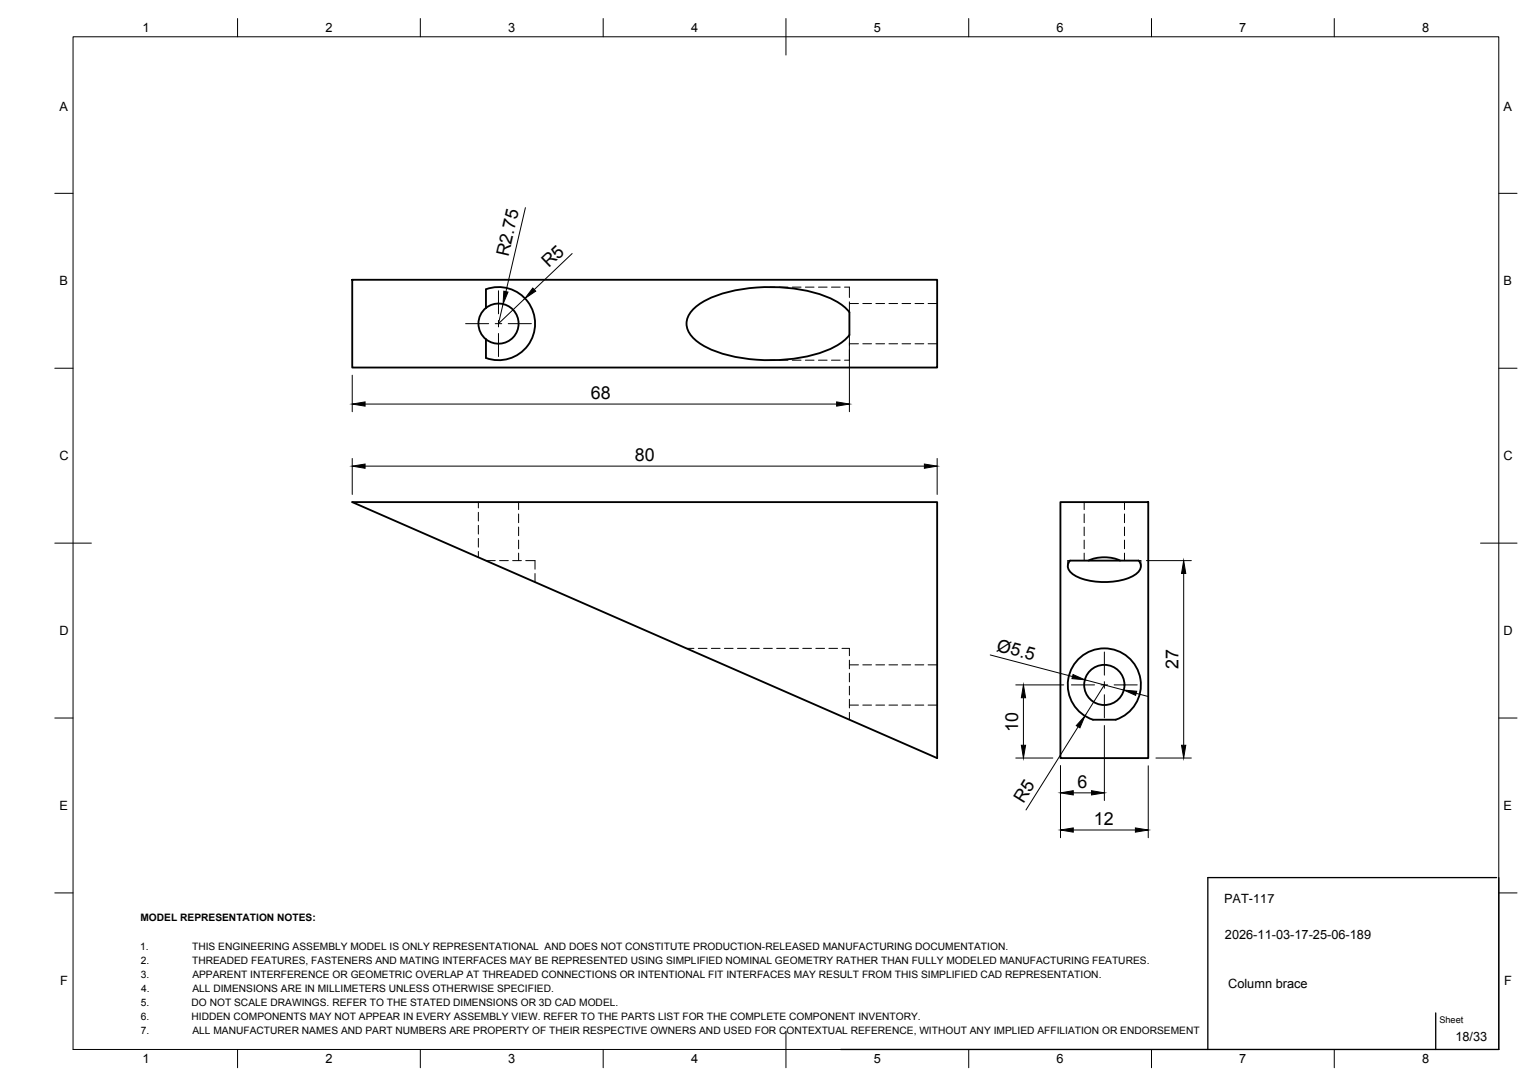
ISO-10303-21;
HEADER;
/* Generated by software containing ST-Developer
 * from STEP Tools, Inc. (www.steptools.com) 
 */

FILE_DESCRIPTION(
/* description */ ('Counterbalanced vertical column'),
/* implementation_level */ '2;1');

FILE_NAME(
/* name */ 'Column brace.step',
/* time_stamp */ '2026-10-29T16:47:22-07:00',
/* author */ (''),
/* organization */ (''),
/* preprocessor_version */ 'ST-DEVELOPER v20.2',
/* originating_system */ 'Autodesk Translation Framework v15.17.0.0',
/* authorisation */ '');

FILE_SCHEMA (('AUTOMOTIVE_DESIGN { 1 0 10303 214 3 1 1 }'));
ENDSEC;

DATA;
#10=MECHANICAL_DESIGN_GEOMETRIC_PRESENTATION_REPRESENTATION('',(#365),#15040);
#270=ELLIPSE('',#7710,0.545757787392906,0.5);
#271=ELLIPSE('',#7716,1.24744637118378,0.5);
#272=ELLIPSE('',#7717,0.300166783066098,0.275);
#295=SHAPE_REPRESENTATION_RELATIONSHIP('SRR','None',#15199,#330);
#330=ADVANCED_BREP_SHAPE_REPRESENTATION('',(#400),#15018);
#365=STYLED_ITEM('',(#15471),#400);
#400=MANIFOLD_SOLID_BREP('Body1',#7088);
#468=FACE_BOUND('',#1400,.T.);
#469=FACE_BOUND('',#1401,.T.);
#470=FACE_BOUND('',#1404,.T.);
#471=FACE_BOUND('',#1408,.T.);
#472=FACE_BOUND('',#1410,.T.);
#605=PLANE('',#7712);
#606=PLANE('',#7715);
#607=PLANE('',#7720);
#608=PLANE('',#7726);
#609=PLANE('',#7727);
#610=PLANE('',#7728);
#611=PLANE('',#7729);
#940=FACE_OUTER_BOUND('',#1397,.T.);
#941=FACE_OUTER_BOUND('',#1398,.T.);
#942=FACE_OUTER_BOUND('',#1399,.T.);
#943=FACE_OUTER_BOUND('',#1402,.T.);
#944=FACE_OUTER_BOUND('',#1403,.T.);
#945=FACE_OUTER_BOUND('',#1405,.T.);
#946=FACE_OUTER_BOUND('',#1406,.T.);
#947=FACE_OUTER_BOUND('',#1407,.T.);
#948=FACE_OUTER_BOUND('',#1409,.T.);
#949=FACE_OUTER_BOUND('',#1411,.T.);
#950=FACE_OUTER_BOUND('',#1412,.T.);
#1397=EDGE_LOOP('',(#5220,#5221));
#1398=EDGE_LOOP('',(#5222,#5223,#5224,#5225,#5226));
#1399=EDGE_LOOP('',(#5227,#5228,#5229,#5230));
#1400=EDGE_LOOP('',(#5231,#5232));
#1401=EDGE_LOOP('',(#5233,#5234,#5235,#5236));
#1402=EDGE_LOOP('',(#5237,#5238,#5239,#5240,#5241,#5242));
#1403=EDGE_LOOP('',(#5243,#5244));
#1404=EDGE_LOOP('',(#5245));
#1405=EDGE_LOOP('',(#5246,#5247));
#1406=EDGE_LOOP('',(#5248,#5249,#5250,#5251));
#1407=EDGE_LOOP('',(#5252,#5253,#5254,#5255));
#1408=EDGE_LOOP('',(#5256));
#1409=EDGE_LOOP('',(#5257,#5258,#5259,#5260));
#1410=EDGE_LOOP('',(#5261));
#1411=EDGE_LOOP('',(#5262,#5263,#5264));
#1412=EDGE_LOOP('',(#5265,#5266,#5267));
#1886=LINE('',#13475,#2557);
#1887=LINE('',#13480,#2558);
#1888=LINE('',#13484,#2559);
#1889=LINE('',#13486,#2560);
#1890=LINE('',#13488,#2561);
#1891=LINE('',#13489,#2562);
#1892=LINE('',#13493,#2563);
#1893=LINE('',#13497,#2564);
#1894=LINE('',#13507,#2565);
#1895=LINE('',#13510,#2566);
#1896=LINE('',#13512,#2567);
#1897=LINE('',#13513,#2568);
#1898=LINE('',#13515,#2569);
#1899=LINE('',#13516,#2570);
#2557=VECTOR('',#8786,1.);
#2558=VECTOR('',#8791,1.);
#2559=VECTOR('',#8794,1.);
#2560=VECTOR('',#8795,1.);
#2561=VECTOR('',#8796,1.);
#2562=VECTOR('',#8797,1.);
#2563=VECTOR('',#8800,1.);
#2564=VECTOR('',#8805,0.275);
#2565=VECTOR('',#8820,0.275);
#2566=VECTOR('',#8823,1.);
#2567=VECTOR('',#8824,1.);
#2568=VECTOR('',#8825,1.);
#2569=VECTOR('',#8828,1.);
#2570=VECTOR('',#8829,1.);
#3173=CIRCLE('',#7711,0.5);
#3174=CIRCLE('',#7713,0.275);
#3175=CIRCLE('',#7714,0.275);
#3176=CIRCLE('',#7719,0.275);
#3177=CIRCLE('',#7721,0.5);
#3178=CIRCLE('',#7722,0.275);
#3179=CIRCLE('',#7725,0.275);
#3450=VERTEX_POINT('',#13469);
#3451=VERTEX_POINT('',#13470);
#3452=VERTEX_POINT('',#13474);
#3453=VERTEX_POINT('',#13476);
#3454=VERTEX_POINT('',#13478);
#3455=VERTEX_POINT('',#13482);
#3456=VERTEX_POINT('',#13483);
#3457=VERTEX_POINT('',#13485);
#3458=VERTEX_POINT('',#13487);
#3459=VERTEX_POINT('',#13490);
#3460=VERTEX_POINT('',#13491);
#3461=VERTEX_POINT('',#13496);
#3462=VERTEX_POINT('',#13501);
#3463=VERTEX_POINT('',#13505);
#3464=VERTEX_POINT('',#13509);
#3465=VERTEX_POINT('',#13511);
#4111=EDGE_CURVE('',#3450,#3451,#270,.T.);
#4112=EDGE_CURVE('',#3450,#3451,#3173,.T.);
#4113=EDGE_CURVE('',#3452,#3450,#1886,.T.);
#4114=EDGE_CURVE('',#3453,#3452,#3174,.T.);
#4115=EDGE_CURVE('',#3454,#3453,#3175,.T.);
#4116=EDGE_CURVE('',#3451,#3454,#1887,.T.);
#4117=EDGE_CURVE('',#3455,#3456,#1888,.T.);
#4118=EDGE_CURVE('',#3455,#3457,#1889,.T.);
#4119=EDGE_CURVE('',#3458,#3457,#1890,.T.);
#4120=EDGE_CURVE('',#3456,#3458,#1891,.T.);
#4121=EDGE_CURVE('',#3459,#3460,#271,.T.);
#4122=EDGE_CURVE('',#3460,#3459,#1892,.T.);
#4123=EDGE_CURVE('',#3454,#3452,#272,.T.);
#4124=EDGE_CURVE('',#3453,#3461,#1893,.T.);
#4125=EDGE_CURVE('',#3461,#3461,#3176,.T.);
#4126=EDGE_CURVE('',#3460,#3459,#3177,.T.);
#4127=EDGE_CURVE('',#3462,#3462,#3178,.T.);
#4128=EDGE_CURVE('',#3463,#3463,#3179,.T.);
#4129=EDGE_CURVE('',#3463,#3462,#1894,.T.);
#4130=EDGE_CURVE('',#3456,#3464,#1895,.T.);
#4131=EDGE_CURVE('',#3465,#3458,#1896,.T.);
#4132=EDGE_CURVE('',#3464,#3465,#1897,.T.);
#4133=EDGE_CURVE('',#3464,#3455,#1898,.T.);
#4134=EDGE_CURVE('',#3457,#3465,#1899,.T.);
#5220=ORIENTED_EDGE('',*,*,#4111,.F.);
#5221=ORIENTED_EDGE('',*,*,#4112,.T.);
#5222=ORIENTED_EDGE('',*,*,#4113,.F.);
#5223=ORIENTED_EDGE('',*,*,#4114,.F.);
#5224=ORIENTED_EDGE('',*,*,#4115,.F.);
#5225=ORIENTED_EDGE('',*,*,#4116,.F.);
#5226=ORIENTED_EDGE('',*,*,#4112,.F.);
#5227=ORIENTED_EDGE('',*,*,#4117,.F.);
#5228=ORIENTED_EDGE('',*,*,#4118,.T.);
#5229=ORIENTED_EDGE('',*,*,#4119,.F.);
#5230=ORIENTED_EDGE('',*,*,#4120,.F.);
#5231=ORIENTED_EDGE('',*,*,#4121,.T.);
#5232=ORIENTED_EDGE('',*,*,#4122,.T.);
#5233=ORIENTED_EDGE('',*,*,#4113,.T.);
#5234=ORIENTED_EDGE('',*,*,#4111,.T.);
#5235=ORIENTED_EDGE('',*,*,#4116,.T.);
#5236=ORIENTED_EDGE('',*,*,#4123,.T.);
#5237=ORIENTED_EDGE('',*,*,#4115,.T.);
#5238=ORIENTED_EDGE('',*,*,#4124,.T.);
#5239=ORIENTED_EDGE('',*,*,#4125,.F.);
#5240=ORIENTED_EDGE('',*,*,#4124,.F.);
#5241=ORIENTED_EDGE('',*,*,#4114,.T.);
#5242=ORIENTED_EDGE('',*,*,#4123,.F.);
#5243=ORIENTED_EDGE('',*,*,#4122,.F.);
#5244=ORIENTED_EDGE('',*,*,#4126,.T.);
#5245=ORIENTED_EDGE('',*,*,#4127,.F.);
#5246=ORIENTED_EDGE('',*,*,#4121,.F.);
#5247=ORIENTED_EDGE('',*,*,#4126,.F.);
#5248=ORIENTED_EDGE('',*,*,#4128,.F.);
#5249=ORIENTED_EDGE('',*,*,#4129,.T.);
#5250=ORIENTED_EDGE('',*,*,#4127,.T.);
#5251=ORIENTED_EDGE('',*,*,#4129,.F.);
#5252=ORIENTED_EDGE('',*,*,#4130,.F.);
#5253=ORIENTED_EDGE('',*,*,#4120,.T.);
#5254=ORIENTED_EDGE('',*,*,#4131,.F.);
#5255=ORIENTED_EDGE('',*,*,#4132,.F.);
#5256=ORIENTED_EDGE('',*,*,#4125,.T.);
#5257=ORIENTED_EDGE('',*,*,#4133,.F.);
#5258=ORIENTED_EDGE('',*,*,#4132,.T.);
#5259=ORIENTED_EDGE('',*,*,#4134,.F.);
#5260=ORIENTED_EDGE('',*,*,#4118,.F.);
#5261=ORIENTED_EDGE('',*,*,#4128,.T.);
#5262=ORIENTED_EDGE('',*,*,#4119,.T.);
#5263=ORIENTED_EDGE('',*,*,#4134,.T.);
#5264=ORIENTED_EDGE('',*,*,#4131,.T.);
#5265=ORIENTED_EDGE('',*,*,#4117,.T.);
#5266=ORIENTED_EDGE('',*,*,#4130,.T.);
#5267=ORIENTED_EDGE('',*,*,#4133,.T.);
#6613=CYLINDRICAL_SURFACE('',#7709,0.5);
#6614=CYLINDRICAL_SURFACE('',#7718,0.275);
#6615=CYLINDRICAL_SURFACE('',#7723,0.5);
#6616=CYLINDRICAL_SURFACE('',#7724,0.275);
#6782=ADVANCED_FACE('',(#940),#6613,.F.);
#6783=ADVANCED_FACE('',(#941),#605,.F.);
#6784=ADVANCED_FACE('',(#942,#468,#469),#606,.T.);
#6785=ADVANCED_FACE('',(#943),#6614,.F.);
#6786=ADVANCED_FACE('',(#944,#470),#607,.T.);
#6787=ADVANCED_FACE('',(#945),#6615,.F.);
#6788=ADVANCED_FACE('',(#946),#6616,.F.);
#6789=ADVANCED_FACE('',(#947,#471),#608,.T.);
#6790=ADVANCED_FACE('',(#948,#472),#609,.T.);
#6791=ADVANCED_FACE('',(#949),#610,.T.);
#6792=ADVANCED_FACE('',(#950),#611,.F.);
#7088=CLOSED_SHELL('',(#6782,#6783,#6784,#6785,#6786,#6787,#6788,#6789,
#6790,#6791,#6792));
#7708=AXIS2_PLACEMENT_3D('',#13467,#8776,#8777);
#7709=AXIS2_PLACEMENT_3D('',#13468,#8778,#8779);
#7710=AXIS2_PLACEMENT_3D('',#13471,#8780,#8781);
#7711=AXIS2_PLACEMENT_3D('',#13472,#8782,#8783);
#7712=AXIS2_PLACEMENT_3D('',#13473,#8784,#8785);
#7713=AXIS2_PLACEMENT_3D('',#13477,#8787,#8788);
#7714=AXIS2_PLACEMENT_3D('',#13479,#8789,#8790);
#7715=AXIS2_PLACEMENT_3D('',#13481,#8792,#8793);
#7716=AXIS2_PLACEMENT_3D('',#13492,#8798,#8799);
#7717=AXIS2_PLACEMENT_3D('',#13494,#8801,#8802);
#7718=AXIS2_PLACEMENT_3D('',#13495,#8803,#8804);
#7719=AXIS2_PLACEMENT_3D('',#13498,#8806,#8807);
#7720=AXIS2_PLACEMENT_3D('',#13499,#8808,#8809);
#7721=AXIS2_PLACEMENT_3D('',#13500,#8810,#8811);
#7722=AXIS2_PLACEMENT_3D('',#13502,#8812,#8813);
#7723=AXIS2_PLACEMENT_3D('',#13503,#8814,#8815);
#7724=AXIS2_PLACEMENT_3D('',#13504,#8816,#8817);
#7725=AXIS2_PLACEMENT_3D('',#13506,#8818,#8819);
#7726=AXIS2_PLACEMENT_3D('',#13508,#8821,#8822);
#7727=AXIS2_PLACEMENT_3D('',#13514,#8826,#8827);
#7728=AXIS2_PLACEMENT_3D('',#13517,#8830,#8831);
#7729=AXIS2_PLACEMENT_3D('',#13518,#8832,#8833);
#8776=DIRECTION('axis',(0.,0.,1.));
#8777=DIRECTION('refdir',(1.,0.,0.));
#8778=DIRECTION('center_axis',(0.,1.,0.));
#8779=DIRECTION('ref_axis',(-1.83697019872103E-16,0.,-1.));
#8780=DIRECTION('center_axis',(0.,0.916157334902189,-0.400818834019708));
#8781=DIRECTION('ref_axis',(0.,-0.400818834019708,-0.916157334902189));
#8782=DIRECTION('center_axis',(0.,1.,0.));
#8783=DIRECTION('ref_axis',(1.,0.,0.));
#8784=DIRECTION('center_axis',(0.,1.,0.));
#8785=DIRECTION('ref_axis',(1.,0.,0.));
#8786=DIRECTION('',(1.,0.,0.));
#8787=DIRECTION('center_axis',(0.,-1.,0.));
#8788=DIRECTION('ref_axis',(1.,0.,0.));
#8789=DIRECTION('center_axis',(0.,-1.,0.));
#8790=DIRECTION('ref_axis',(1.,0.,0.));
#8791=DIRECTION('',(1.,0.,0.));
#8792=DIRECTION('center_axis',(0.,-0.916157334902189,0.400818834019708));
#8793=DIRECTION('ref_axis',(0.,-0.400818834019708,-0.916157334902189));
#8794=DIRECTION('',(0.,0.400818834019708,0.916157334902189));
#8795=DIRECTION('',(1.,0.,0.));
#8796=DIRECTION('',(0.,-0.400818834019708,-0.916157334902189));
#8797=DIRECTION('',(1.,0.,0.));
#8798=DIRECTION('center_axis',(0.,0.916157334902189,-0.400818834019708));
#8799=DIRECTION('ref_axis',(0.,0.400818834019708,0.916157334902189));
#8800=DIRECTION('',(-1.,0.,0.));
#8801=DIRECTION('center_axis',(0.,0.916157334902189,-0.400818834019708));
#8802=DIRECTION('ref_axis',(0.,-0.400818834019708,-0.916157334902189));
#8803=DIRECTION('center_axis',(0.,1.,0.));
#8804=DIRECTION('ref_axis',(1.,0.,0.));
#8805=DIRECTION('',(0.,1.,0.));
#8806=DIRECTION('center_axis',(0.,-1.,0.));
#8807=DIRECTION('ref_axis',(1.,0.,0.));
#8808=DIRECTION('center_axis',(0.,0.,1.));
#8809=DIRECTION('ref_axis',(1.,0.,0.));
#8810=DIRECTION('center_axis',(0.,0.,1.));
#8811=DIRECTION('ref_axis',(1.,0.,0.));
#8812=DIRECTION('center_axis',(0.,0.,1.));
#8813=DIRECTION('ref_axis',(1.,0.,0.));
#8814=DIRECTION('center_axis',(0.,0.,1.));
#8815=DIRECTION('ref_axis',(6.12323399573677E-17,1.,0.));
#8816=DIRECTION('center_axis',(0.,0.,1.));
#8817=DIRECTION('ref_axis',(1.,0.,0.));
#8818=DIRECTION('center_axis',(0.,0.,1.));
#8819=DIRECTION('ref_axis',(1.,0.,0.));
#8820=DIRECTION('',(0.,0.,1.));
#8821=DIRECTION('center_axis',(0.,1.,0.));
#8822=DIRECTION('ref_axis',(0.,0.,1.));
#8823=DIRECTION('',(0.,0.,-1.));
#8824=DIRECTION('',(0.,0.,1.));
#8825=DIRECTION('',(1.,0.,0.));
#8826=DIRECTION('center_axis',(0.,0.,-1.));
#8827=DIRECTION('ref_axis',(0.,1.,0.));
#8828=DIRECTION('',(0.,-1.,0.));
#8829=DIRECTION('',(0.,1.,0.));
#8830=DIRECTION('center_axis',(1.,0.,0.));
#8831=DIRECTION('ref_axis',(0.,0.,-1.));
#8832=DIRECTION('center_axis',(1.,0.,0.));
#8833=DIRECTION('ref_axis',(0.,0.,-1.));
#13467=CARTESIAN_POINT('',(0.,0.,0.));
#13468=CARTESIAN_POINT('Origin',(3.,-2.6,6.));
#13469=CARTESIAN_POINT('',(3.46969377779353,-1.8,6.17142857142857));
#13470=CARTESIAN_POINT('',(2.53030622220647,-1.8,6.17142857142857));
#13471=CARTESIAN_POINT('Origin',(3.,-1.875,6.));
#13472=CARTESIAN_POINT('Origin',(3.,-1.8,6.));
#13473=CARTESIAN_POINT('Origin',(3.,-1.8,6.));
#13474=CARTESIAN_POINT('',(3.21502847462129,-1.8,6.17142857142857));
#13475=CARTESIAN_POINT('',(2.7,-1.8,6.17142857142857));
#13476=CARTESIAN_POINT('',(2.725,-1.8,6.));
#13477=CARTESIAN_POINT('Origin',(3.,-1.8,6.));
#13478=CARTESIAN_POINT('',(2.78497152537871,-1.8,6.17142857142857));
#13479=CARTESIAN_POINT('Origin',(3.,-1.8,6.));
#13480=CARTESIAN_POINT('',(2.7,-1.8,6.17142857142857));
#13481=CARTESIAN_POINT('Origin',(2.4,-1.,8.));
#13482=CARTESIAN_POINT('',(2.4,-4.5,0.));
#13483=CARTESIAN_POINT('',(2.4,-1.,8.));
#13484=CARTESIAN_POINT('',(2.4,-4.5,0.));
#13485=CARTESIAN_POINT('',(3.6,-4.5,0.));
#13486=CARTESIAN_POINT('',(2.4,-4.5,0.));
#13487=CARTESIAN_POINT('',(3.6,-1.,8.));
#13488=CARTESIAN_POINT('',(3.6,-4.5,0.));
#13489=CARTESIAN_POINT('',(2.4,-1.,8.));
#13490=CARTESIAN_POINT('',(2.84387505004004,-3.975,1.2));
#13491=CARTESIAN_POINT('',(3.15612494995996,-3.975,1.2));
#13492=CARTESIAN_POINT('Origin',(3.,-3.5,2.28571428571429));
#13493=CARTESIAN_POINT('',(2.7,-3.975,1.2));
#13494=CARTESIAN_POINT('Origin',(3.,-1.875,6.));
#13495=CARTESIAN_POINT('Origin',(3.,-2.6,6.));
#13496=CARTESIAN_POINT('',(2.725,-1.,6.));
#13497=CARTESIAN_POINT('',(2.725,-2.6,6.));
#13498=CARTESIAN_POINT('Origin',(3.,-1.,6.));
#13499=CARTESIAN_POINT('Origin',(3.,-3.5,1.2));
#13500=CARTESIAN_POINT('Origin',(3.,-3.5,1.2));
#13501=CARTESIAN_POINT('',(2.725,-3.5,1.2));
#13502=CARTESIAN_POINT('Origin',(3.,-3.5,1.2));
#13503=CARTESIAN_POINT('Origin',(3.,-3.5,1.2));
#13504=CARTESIAN_POINT('Origin',(3.,-3.5,-0.1));
#13505=CARTESIAN_POINT('',(2.725,-3.5,0.));
#13506=CARTESIAN_POINT('Origin',(3.,-3.5,0.));
#13507=CARTESIAN_POINT('',(2.725,-3.5,-0.1));
#13508=CARTESIAN_POINT('Origin',(2.4,-1.,0.));
#13509=CARTESIAN_POINT('',(2.4,-1.,0.));
#13510=CARTESIAN_POINT('',(2.4,-1.,8.));
#13511=CARTESIAN_POINT('',(3.6,-1.,0.));
#13512=CARTESIAN_POINT('',(3.6,-1.,8.));
#13513=CARTESIAN_POINT('',(2.4,-1.,0.));
#13514=CARTESIAN_POINT('Origin',(2.4,-4.5,0.));
#13515=CARTESIAN_POINT('',(2.4,-1.,0.));
#13516=CARTESIAN_POINT('',(3.6,-1.,0.));
#13517=CARTESIAN_POINT('Origin',(3.6,-2.75,4.));
#13518=CARTESIAN_POINT('Origin',(2.4,-2.75,4.));
#14978=UNCERTAINTY_MEASURE_WITH_UNIT(LENGTH_MEASURE(0.001),#15041,
'DISTANCE_ACCURACY_VALUE',
'Maximum model space distance between geometric entities at asserted c
onnectivities');
#15000=UNCERTAINTY_MEASURE_WITH_UNIT(LENGTH_MEASURE(0.001),#15041,
'DISTANCE_ACCURACY_VALUE',
'Maximum model space distance between geometric entities at asserted c
onnectivities');
#15018=(
GEOMETRIC_REPRESENTATION_CONTEXT(3)
GLOBAL_UNCERTAINTY_ASSIGNED_CONTEXT((#14978))
GLOBAL_UNIT_ASSIGNED_CONTEXT((#15041,#15043,#15044))
REPRESENTATION_CONTEXT('','3D')
);
#15040=(
GEOMETRIC_REPRESENTATION_CONTEXT(3)
GLOBAL_UNCERTAINTY_ASSIGNED_CONTEXT((#15000))
GLOBAL_UNIT_ASSIGNED_CONTEXT((#15041,#15043,#15044))
REPRESENTATION_CONTEXT('','3D')
);
#15041=(
LENGTH_UNIT()
NAMED_UNIT(*)
SI_UNIT(.CENTI.,.METRE.)
);
#15043=(
NAMED_UNIT(*)
PLANE_ANGLE_UNIT()
SI_UNIT($,.RADIAN.)
);
#15044=(
NAMED_UNIT(*)
SI_UNIT($,.STERADIAN.)
SOLID_ANGLE_UNIT()
);
#15062=SHAPE_DEFINITION_REPRESENTATION(#15101,#15199);
#15101=PRODUCT_DEFINITION_SHAPE('',$,#15239);
#15199=SHAPE_REPRESENTATION('',(#7708),#15018);
#15221=PRODUCT_DEFINITION_CONTEXT('part definition',#15340,'design');
#15239=PRODUCT_DEFINITION('Column brace','Column brace',#15278,#15221);
#15278=PRODUCT_DEFINITION_FORMATION('',$,#15359);
#15340=APPLICATION_CONTEXT(
'Core Data for Automotive Mechanical Design Process');
#15341=PRODUCT_CONTEXT('part definition',#15340,'mechanical');
#15359=PRODUCT('Column brace','Column brace','Column brace',(#15341));
#15465=COLOUR_RGB('Off White',0.89,0.88,0.83);
#15466=FILL_AREA_STYLE_COLOUR('',#15465);
#15467=FILL_AREA_STYLE('',(#15466));
#15468=SURFACE_STYLE_FILL_AREA(#15467);
#15469=SURFACE_SIDE_STYLE('',(#15468));
#15470=SURFACE_STYLE_USAGE(.BOTH.,#15469);
#15471=PRESENTATION_STYLE_ASSIGNMENT((#15470));
ENDSEC;
END-ISO-10303-21;
